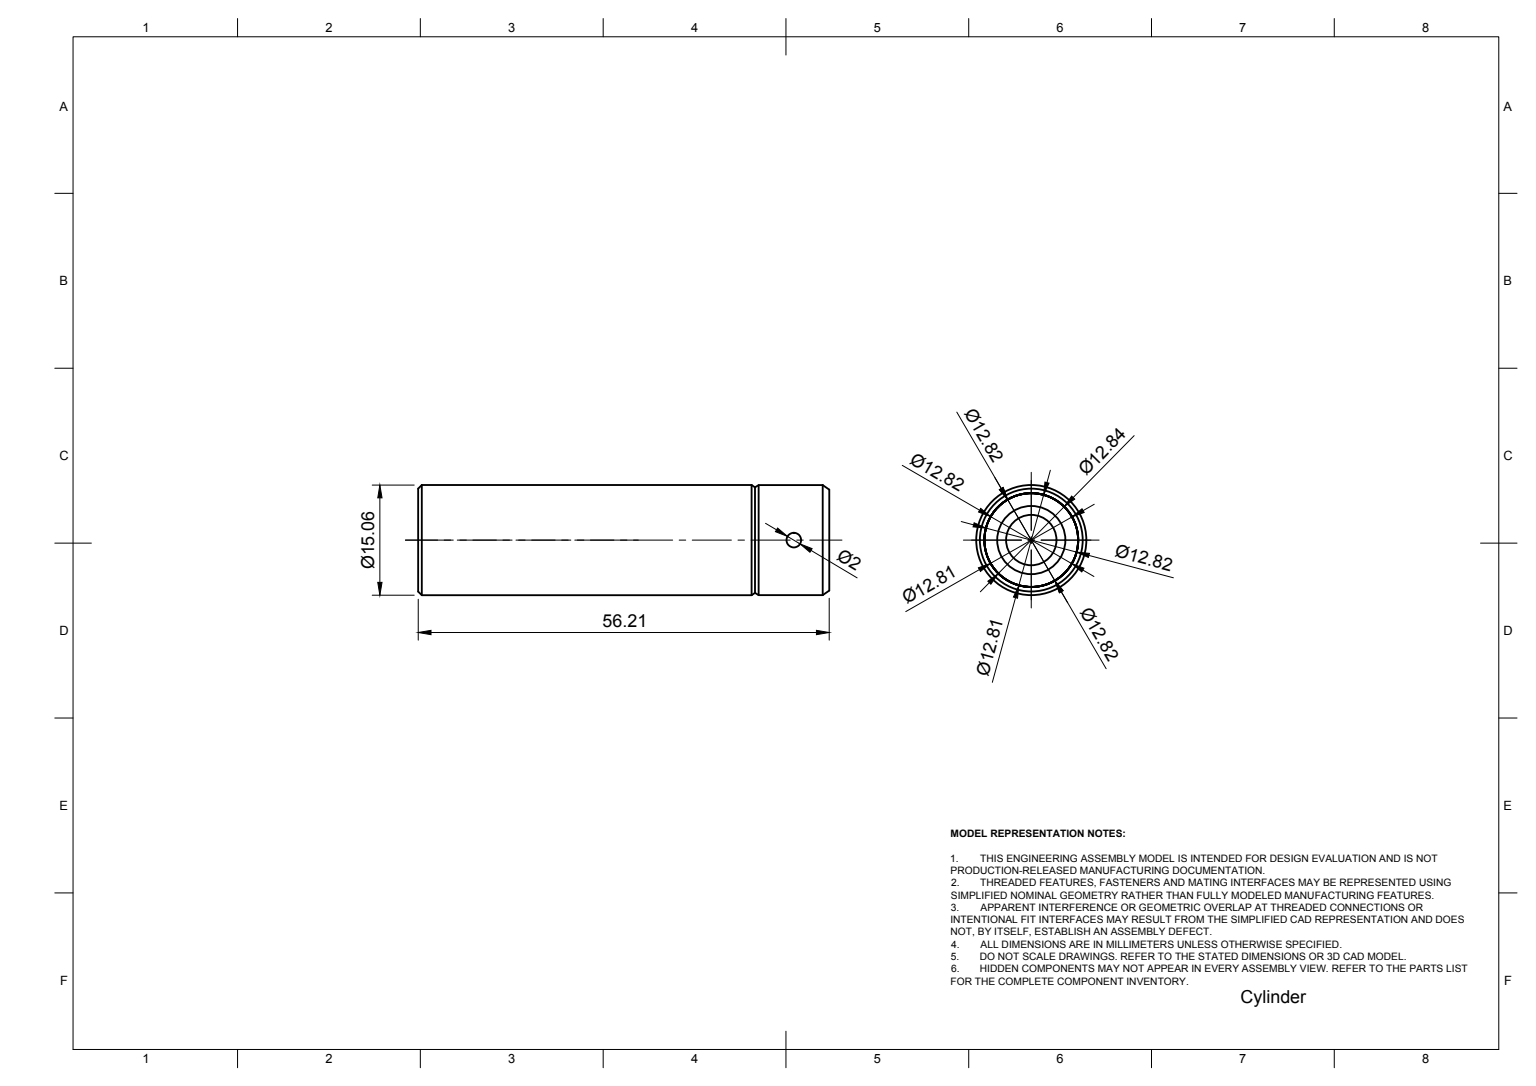
ISO-10303-21;
HEADER;
/* Generated by software containing ST-Developer
 * from STEP Tools, Inc. (www.steptools.com) 
 */

FILE_DESCRIPTION(
/* description */ (''),
/* implementation_level */ '2;1');

FILE_NAME(
/* name */ 'Cylinder.step',
/* time_stamp */ '2026-10-06T13:15:55-07:00',
/* author */ (''),
/* organization */ (''),
/* preprocessor_version */ 'ST-DEVELOPER v20.2',
/* originating_system */ 'Autodesk Translation Framework v15.15.0.0',
/* authorisation */ '');

FILE_SCHEMA (('AUTOMOTIVE_DESIGN { 1 0 10303 214 3 1 1 }'));
ENDSEC;

DATA;
#10=MECHANICAL_DESIGN_GEOMETRIC_PRESENTATION_REPRESENTATION('',(#114),#27707);
#73=CONICAL_SURFACE('',#4093,7.27835105742136,0.785398163397451);
#74=CONICAL_SURFACE('',#4106,7.20746054905241,0.610790367386849);
#75=CONICAL_SURFACE('',#4111,7.36529369971832,0.557210682142491);
#76=CONICAL_SURFACE('',#4113,7.36790580323689,0.610790367386849);
#77=CONICAL_SURFACE('',#4114,6.41628586403442,0.000295609290232646);
#78=CONICAL_SURFACE('',#4118,6.40906719549494,0.00029560929023293);
#79=CONICAL_SURFACE('',#4126,6.40820475053297,0.000295609290233083);
#80=CONICAL_SURFACE('',#4130,6.40732538114918,0.000295609290232334);
#81=CONICAL_SURFACE('',#4134,6.40667124022599,0.000295609290231853);
#94=SHAPE_REPRESENTATION_RELATIONSHIP('SRR','None',#27751,#104);
#104=ADVANCED_BREP_SHAPE_REPRESENTATION('',(#124),#27703);
#114=STYLED_ITEM('',(#27804),#124);
#124=MANIFOLD_SOLID_BREP('Body1',#3840);
#142=FACE_BOUND('',#796,.T.);
#143=FACE_BOUND('',#801,.T.);
#144=FACE_BOUND('',#804,.T.);
#145=FACE_BOUND('',#811,.T.);
#146=FACE_BOUND('',#814,.T.);
#147=FACE_BOUND('',#821,.T.);
#148=FACE_BOUND('',#824,.T.);
#149=FACE_BOUND('',#826,.T.);
#150=FACE_BOUND('',#828,.T.);
#194=PLANE('',#4096);
#195=PLANE('',#4104);
#196=PLANE('',#4120);
#197=PLANE('',#4124);
#198=PLANE('',#4136);
#199=PLANE('',#4140);
#200=PLANE('',#4143);
#260=CIRCLE('',#4094,7.52835105742136);
#261=CIRCLE('',#4095,7.02835105742136);
#262=CIRCLE('',#4097,6.42021067919505);
#263=CIRCLE('',#4099,7.52835105742136);
#264=CIRCLE('',#4102,5.);
#265=CIRCLE('',#4103,5.);
#266=CIRCLE('',#4105,3.44589712386029);
#267=CIRCLE('',#4107,7.52312685038423);
#268=CIRCLE('',#4108,6.89179424772059);
#269=CIRCLE('',#4110,7.52312685038423);
#270=CIRCLE('',#4112,7.20746054905241);
#271=CIRCLE('',#4115,6.40969108660508);
#272=CIRCLE('',#4117,6.40969108660508);
#273=CIRCLE('',#4119,6.40881029802658);
#274=CIRCLE('',#4121,6.41550316824698);
#275=CIRCLE('',#4123,6.41550316824698);
#276=CIRCLE('',#4125,6.40853872070288);
#277=CIRCLE('',#4127,6.40787078036307);
#278=CIRCLE('',#4129,6.40787078036307);
#279=CIRCLE('',#4131,6.40706623219228);
#280=CIRCLE('',#4133,6.40706623219228);
#281=CIRCLE('',#4135,6.4065967297173);
#282=CIRCLE('',#4137,4.66385643997278);
#283=CIRCLE('',#4139,4.66385643997278);
#284=CIRCLE('',#4141,3.44589712386029);
#393=CYLINDRICAL_SURFACE('',#4098,7.52835105742136);
#394=CYLINDRICAL_SURFACE('',#4100,0.999999999999999);
#395=CYLINDRICAL_SURFACE('',#4101,5.);
#396=CYLINDRICAL_SURFACE('',#4109,7.52312685038423);
#397=CYLINDRICAL_SURFACE('',#4116,6.40969108660508);
#398=CYLINDRICAL_SURFACE('',#4122,6.41550316824698);
#399=CYLINDRICAL_SURFACE('',#4128,6.40787078036307);
#400=CYLINDRICAL_SURFACE('',#4132,6.40706623219228);
#401=CYLINDRICAL_SURFACE('',#4138,4.66385643997278);
#402=CYLINDRICAL_SURFACE('',#4142,3.44589712386029);
#559=FACE_OUTER_BOUND('',#794,.T.);
#560=FACE_OUTER_BOUND('',#795,.T.);
#561=FACE_OUTER_BOUND('',#797,.T.);
#562=FACE_OUTER_BOUND('',#798,.T.);
#563=FACE_OUTER_BOUND('',#799,.T.);
#564=FACE_OUTER_BOUND('',#800,.T.);
#565=FACE_OUTER_BOUND('',#802,.T.);
#566=FACE_OUTER_BOUND('',#803,.T.);
#567=FACE_OUTER_BOUND('',#805,.T.);
#568=FACE_OUTER_BOUND('',#806,.T.);
#569=FACE_OUTER_BOUND('',#807,.T.);
#570=FACE_OUTER_BOUND('',#808,.T.);
#571=FACE_OUTER_BOUND('',#809,.T.);
#572=FACE_OUTER_BOUND('',#810,.T.);
#573=FACE_OUTER_BOUND('',#812,.T.);
#574=FACE_OUTER_BOUND('',#813,.T.);
#575=FACE_OUTER_BOUND('',#815,.T.);
#576=FACE_OUTER_BOUND('',#816,.T.);
#577=FACE_OUTER_BOUND('',#817,.T.);
#578=FACE_OUTER_BOUND('',#818,.T.);
#579=FACE_OUTER_BOUND('',#819,.T.);
#580=FACE_OUTER_BOUND('',#820,.T.);
#581=FACE_OUTER_BOUND('',#822,.T.);
#582=FACE_OUTER_BOUND('',#823,.T.);
#583=FACE_OUTER_BOUND('',#825,.T.);
#584=FACE_OUTER_BOUND('',#827,.T.);
#794=EDGE_LOOP('',(#3123,#3124,#3125,#3126));
#795=EDGE_LOOP('',(#3127));
#796=EDGE_LOOP('',(#3128));
#797=EDGE_LOOP('',(#3129,#3130,#3131,#3132));
#798=EDGE_LOOP('',(#3133,#3134,#3135,#3136,#3137,#3138));
#799=EDGE_LOOP('',(#3139,#3140,#3141,#3142));
#800=EDGE_LOOP('',(#3143));
#801=EDGE_LOOP('',(#3144));
#802=EDGE_LOOP('',(#3145,#3146,#3147,#3148));
#803=EDGE_LOOP('',(#3149,#3150,#3151,#3152));
#804=EDGE_LOOP('',(#3153,#3154));
#805=EDGE_LOOP('',(#3155,#3156,#3157,#3158));
#806=EDGE_LOOP('',(#3159,#3160,#3161,#3162));
#807=EDGE_LOOP('',(#3163,#3164,#3165,#3166));
#808=EDGE_LOOP('',(#3167,#3168,#3169,#3170));
#809=EDGE_LOOP('',(#3171,#3172,#3173,#3174));
#810=EDGE_LOOP('',(#3175));
#811=EDGE_LOOP('',(#3176));
#812=EDGE_LOOP('',(#3177,#3178,#3179,#3180));
#813=EDGE_LOOP('',(#3181));
#814=EDGE_LOOP('',(#3182));
#815=EDGE_LOOP('',(#3183,#3184,#3185,#3186));
#816=EDGE_LOOP('',(#3187,#3188,#3189,#3190));
#817=EDGE_LOOP('',(#3191,#3192,#3193,#3194));
#818=EDGE_LOOP('',(#3195,#3196,#3197,#3198));
#819=EDGE_LOOP('',(#3199,#3200,#3201,#3202));
#820=EDGE_LOOP('',(#3203));
#821=EDGE_LOOP('',(#3204));
#822=EDGE_LOOP('',(#3205,#3206,#3207,#3208));
#823=EDGE_LOOP('',(#3209));
#824=EDGE_LOOP('',(#3210));
#825=EDGE_LOOP('',(#3211,#3212,#3213,#3214));
#826=EDGE_LOOP('',(#3215,#3216));
#827=EDGE_LOOP('',(#3217));
#828=EDGE_LOOP('',(#3218));
#1032=LINE('',#15534,#1208);
#1033=LINE('',#15541,#1209);
#1034=LINE('',#15583,#1210);
#1035=LINE('',#15625,#1211);
#1036=LINE('',#15634,#1212);
#1037=LINE('',#15639,#1213);
#1038=LINE('',#15642,#1214);
#1039=LINE('',#15645,#1215);
#1040=LINE('',#15649,#1216);
#1041=LINE('',#15653,#1217);
#1042=LINE('',#15657,#1218);
#1043=LINE('',#15664,#1219);
#1044=LINE('',#15671,#1220);
#1045=LINE('',#15675,#1221);
#1046=LINE('',#15679,#1222);
#1047=LINE('',#15683,#1223);
#1048=LINE('',#15687,#1224);
#1049=LINE('',#15694,#1225);
#1050=LINE('',#15699,#1226);
#1208=VECTOR('',#4685,7.27835105742136);
#1209=VECTOR('',#4694,7.52835105742136);
#1210=VECTOR('',#4699,0.999999999999999);
#1211=VECTOR('',#4704,5.);
#1212=VECTOR('',#4715,7.20746054905241);
#1213=VECTOR('',#4722,7.52312685038423);
#1214=VECTOR('',#4725,7.36529369971832);
#1215=VECTOR('',#4730,7.36790580323689);
#1216=VECTOR('',#4735,6.41628586403442);
#1217=VECTOR('',#4740,6.40969108660508);
#1218=VECTOR('',#4745,6.40906719549494);
#1219=VECTOR('',#4754,6.41550316824698);
#1220=VECTOR('',#4763,6.40820475053297);
#1221=VECTOR('',#4768,6.40787078036307);
#1222=VECTOR('',#4773,6.40732538114918);
#1223=VECTOR('',#4778,6.40706623219228);
#1224=VECTOR('',#4783,6.40667124022599);
#1225=VECTOR('',#4792,4.66385643997278);
#1226=VECTOR('',#4799,3.44589712386029);
#1438=B_SPLINE_CURVE_WITH_KNOTS('',3,(#15546,#15547,#15548,#15549,#15550,
#15551,#15552,#15553,#15554,#15555,#15556,#15557,#15558,#15559,#15560,#15561,
#15562,#15563,#15564,#15565,#15566,#15567,#15568,#15569,#15570,#15571),
 .UNSPECIFIED.,.F.,.F.,(4,2,2,2,2,2,2,2,2,2,2,2,4),(-0.606481282784619,
-0.568571286664201,-0.530661290543783,-0.492761126316124,-0.454860962088464,
-0.416960797860805,-0.379060633633146,-0.341150637512728,-0.30324064139231,
-0.265330645271891,-0.227420649151473,-0.189520484923814,-0.151620320696155),
 .UNSPECIFIED.);
#1439=B_SPLINE_CURVE_WITH_KNOTS('',3,(#15572,#15573,#15574,#15575,#15576,
#15577,#15578,#15579,#15580,#15581),.UNSPECIFIED.,.F.,.F.,(4,2,2,2,4),(-0.151620320696155,
-0.113720156468496,-0.0758199922408364,-0.0379099961204182,0.),
 .UNSPECIFIED.);
#1440=B_SPLINE_CURVE_WITH_KNOTS('',3,(#15585,#15586,#15587,#15588,#15589,
#15590,#15591,#15592,#15593,#15594),.UNSPECIFIED.,.F.,.F.,(4,2,2,2,4),(0.,
0.0377168406459521,0.0754336812919042,0.113150118256495,0.150866555221085),
 .UNSPECIFIED.);
#1441=B_SPLINE_CURVE_WITH_KNOTS('',3,(#15595,#15596,#15597,#15598,#15599,
#15600,#15601,#15602,#15603,#15604,#15605,#15606,#15607,#15608,#15609,#15610,
#15611,#15612,#15613,#15614,#15615,#15616,#15617,#15618,#15619,#15620),
 .UNSPECIFIED.,.F.,.F.,(4,2,2,2,2,2,2,2,2,2,2,2,4),(0.150866555221085,0.188582992185676,
0.226299429150267,0.264016269796219,0.301733110442171,0.339449951088123,
0.377166791734075,0.414883228698666,0.452599665663256,0.490316102627847,
0.528032539592437,0.565749380238389,0.603466220884342),.UNSPECIFIED.);
#1749=VERTEX_POINT('',#15531);
#1750=VERTEX_POINT('',#15533);
#1751=VERTEX_POINT('',#15537);
#1752=VERTEX_POINT('',#15540);
#1753=VERTEX_POINT('',#15544);
#1754=VERTEX_POINT('',#15545);
#1755=VERTEX_POINT('',#15582);
#1756=VERTEX_POINT('',#15584);
#1757=VERTEX_POINT('',#15622);
#1758=VERTEX_POINT('',#15624);
#1759=VERTEX_POINT('',#15628);
#1760=VERTEX_POINT('',#15631);
#1761=VERTEX_POINT('',#15633);
#1762=VERTEX_POINT('',#15637);
#1763=VERTEX_POINT('',#15641);
#1764=VERTEX_POINT('',#15647);
#1765=VERTEX_POINT('',#15651);
#1766=VERTEX_POINT('',#15655);
#1767=VERTEX_POINT('',#15659);
#1768=VERTEX_POINT('',#15662);
#1769=VERTEX_POINT('',#15666);
#1770=VERTEX_POINT('',#15669);
#1771=VERTEX_POINT('',#15673);
#1772=VERTEX_POINT('',#15677);
#1773=VERTEX_POINT('',#15681);
#1774=VERTEX_POINT('',#15685);
#1775=VERTEX_POINT('',#15689);
#1776=VERTEX_POINT('',#15692);
#1777=VERTEX_POINT('',#15696);
#2231=EDGE_CURVE('',#1749,#1749,#260,.T.);
#2232=EDGE_CURVE('',#1749,#1750,#1032,.T.);
#2233=EDGE_CURVE('',#1750,#1750,#261,.T.);
#2234=EDGE_CURVE('',#1751,#1751,#262,.T.);
#2235=EDGE_CURVE('',#1749,#1752,#1033,.T.);
#2236=EDGE_CURVE('',#1752,#1752,#263,.T.);
#2237=EDGE_CURVE('',#1753,#1754,#1438,.T.);
#2238=EDGE_CURVE('',#1754,#1753,#1439,.T.);
#2239=EDGE_CURVE('',#1754,#1755,#1034,.T.);
#2240=EDGE_CURVE('',#1756,#1755,#1440,.T.);
#2241=EDGE_CURVE('',#1755,#1756,#1441,.T.);
#2242=EDGE_CURVE('',#1757,#1757,#264,.T.);
#2243=EDGE_CURVE('',#1757,#1758,#1035,.T.);
#2244=EDGE_CURVE('',#1758,#1758,#265,.T.);
#2245=EDGE_CURVE('',#1759,#1759,#266,.T.);
#2246=EDGE_CURVE('',#1760,#1760,#267,.T.);
#2247=EDGE_CURVE('',#1760,#1761,#1036,.T.);
#2248=EDGE_CURVE('',#1761,#1761,#268,.T.);
#2249=EDGE_CURVE('',#1762,#1762,#269,.T.);
#2250=EDGE_CURVE('',#1762,#1760,#1037,.T.);
#2251=EDGE_CURVE('',#1762,#1763,#1038,.T.);
#2252=EDGE_CURVE('',#1763,#1763,#270,.T.);
#2253=EDGE_CURVE('',#1752,#1763,#1039,.T.);
#2254=EDGE_CURVE('',#1764,#1764,#271,.T.);
#2255=EDGE_CURVE('',#1764,#1751,#1040,.T.);
#2256=EDGE_CURVE('',#1765,#1765,#272,.T.);
#2257=EDGE_CURVE('',#1765,#1764,#1041,.T.);
#2258=EDGE_CURVE('',#1766,#1766,#273,.T.);
#2259=EDGE_CURVE('',#1766,#1765,#1042,.T.);
#2260=EDGE_CURVE('',#1767,#1767,#274,.T.);
#2261=EDGE_CURVE('',#1768,#1768,#275,.T.);
#2262=EDGE_CURVE('',#1768,#1767,#1043,.T.);
#2263=EDGE_CURVE('',#1769,#1769,#276,.T.);
#2264=EDGE_CURVE('',#1770,#1770,#277,.T.);
#2265=EDGE_CURVE('',#1770,#1769,#1044,.T.);
#2266=EDGE_CURVE('',#1771,#1771,#278,.T.);
#2267=EDGE_CURVE('',#1771,#1770,#1045,.T.);
#2268=EDGE_CURVE('',#1772,#1772,#279,.T.);
#2269=EDGE_CURVE('',#1772,#1771,#1046,.T.);
#2270=EDGE_CURVE('',#1773,#1773,#280,.T.);
#2271=EDGE_CURVE('',#1773,#1772,#1047,.T.);
#2272=EDGE_CURVE('',#1774,#1774,#281,.T.);
#2273=EDGE_CURVE('',#1774,#1773,#1048,.T.);
#2274=EDGE_CURVE('',#1775,#1775,#282,.T.);
#2275=EDGE_CURVE('',#1776,#1776,#283,.T.);
#2276=EDGE_CURVE('',#1776,#1775,#1049,.T.);
#2277=EDGE_CURVE('',#1777,#1777,#284,.T.);
#2278=EDGE_CURVE('',#1759,#1777,#1050,.T.);
#3123=ORIENTED_EDGE('',*,*,#2231,.T.);
#3124=ORIENTED_EDGE('',*,*,#2232,.T.);
#3125=ORIENTED_EDGE('',*,*,#2233,.T.);
#3126=ORIENTED_EDGE('',*,*,#2232,.F.);
#3127=ORIENTED_EDGE('',*,*,#2233,.F.);
#3128=ORIENTED_EDGE('',*,*,#2234,.F.);
#3129=ORIENTED_EDGE('',*,*,#2231,.F.);
#3130=ORIENTED_EDGE('',*,*,#2235,.T.);
#3131=ORIENTED_EDGE('',*,*,#2236,.T.);
#3132=ORIENTED_EDGE('',*,*,#2235,.F.);
#3133=ORIENTED_EDGE('',*,*,#2237,.F.);
#3134=ORIENTED_EDGE('',*,*,#2238,.F.);
#3135=ORIENTED_EDGE('',*,*,#2239,.T.);
#3136=ORIENTED_EDGE('',*,*,#2240,.F.);
#3137=ORIENTED_EDGE('',*,*,#2241,.F.);
#3138=ORIENTED_EDGE('',*,*,#2239,.F.);
#3139=ORIENTED_EDGE('',*,*,#2242,.F.);
#3140=ORIENTED_EDGE('',*,*,#2243,.T.);
#3141=ORIENTED_EDGE('',*,*,#2244,.T.);
#3142=ORIENTED_EDGE('',*,*,#2243,.F.);
#3143=ORIENTED_EDGE('',*,*,#2244,.F.);
#3144=ORIENTED_EDGE('',*,*,#2245,.T.);
#3145=ORIENTED_EDGE('',*,*,#2246,.F.);
#3146=ORIENTED_EDGE('',*,*,#2247,.T.);
#3147=ORIENTED_EDGE('',*,*,#2248,.T.);
#3148=ORIENTED_EDGE('',*,*,#2247,.F.);
#3149=ORIENTED_EDGE('',*,*,#2249,.F.);
#3150=ORIENTED_EDGE('',*,*,#2250,.T.);
#3151=ORIENTED_EDGE('',*,*,#2246,.T.);
#3152=ORIENTED_EDGE('',*,*,#2250,.F.);
#3153=ORIENTED_EDGE('',*,*,#2240,.T.);
#3154=ORIENTED_EDGE('',*,*,#2241,.T.);
#3155=ORIENTED_EDGE('',*,*,#2249,.T.);
#3156=ORIENTED_EDGE('',*,*,#2251,.T.);
#3157=ORIENTED_EDGE('',*,*,#2252,.F.);
#3158=ORIENTED_EDGE('',*,*,#2251,.F.);
#3159=ORIENTED_EDGE('',*,*,#2236,.F.);
#3160=ORIENTED_EDGE('',*,*,#2253,.T.);
#3161=ORIENTED_EDGE('',*,*,#2252,.T.);
#3162=ORIENTED_EDGE('',*,*,#2253,.F.);
#3163=ORIENTED_EDGE('',*,*,#2254,.F.);
#3164=ORIENTED_EDGE('',*,*,#2255,.T.);
#3165=ORIENTED_EDGE('',*,*,#2234,.T.);
#3166=ORIENTED_EDGE('',*,*,#2255,.F.);
#3167=ORIENTED_EDGE('',*,*,#2256,.F.);
#3168=ORIENTED_EDGE('',*,*,#2257,.T.);
#3169=ORIENTED_EDGE('',*,*,#2254,.T.);
#3170=ORIENTED_EDGE('',*,*,#2257,.F.);
#3171=ORIENTED_EDGE('',*,*,#2258,.F.);
#3172=ORIENTED_EDGE('',*,*,#2259,.T.);
#3173=ORIENTED_EDGE('',*,*,#2256,.T.);
#3174=ORIENTED_EDGE('',*,*,#2259,.F.);
#3175=ORIENTED_EDGE('',*,*,#2260,.F.);
#3176=ORIENTED_EDGE('',*,*,#2258,.T.);
#3177=ORIENTED_EDGE('',*,*,#2261,.F.);
#3178=ORIENTED_EDGE('',*,*,#2262,.T.);
#3179=ORIENTED_EDGE('',*,*,#2260,.T.);
#3180=ORIENTED_EDGE('',*,*,#2262,.F.);
#3181=ORIENTED_EDGE('',*,*,#2261,.T.);
#3182=ORIENTED_EDGE('',*,*,#2263,.F.);
#3183=ORIENTED_EDGE('',*,*,#2264,.F.);
#3184=ORIENTED_EDGE('',*,*,#2265,.T.);
#3185=ORIENTED_EDGE('',*,*,#2263,.T.);
#3186=ORIENTED_EDGE('',*,*,#2265,.F.);
#3187=ORIENTED_EDGE('',*,*,#2266,.F.);
#3188=ORIENTED_EDGE('',*,*,#2267,.T.);
#3189=ORIENTED_EDGE('',*,*,#2264,.T.);
#3190=ORIENTED_EDGE('',*,*,#2267,.F.);
#3191=ORIENTED_EDGE('',*,*,#2268,.F.);
#3192=ORIENTED_EDGE('',*,*,#2269,.T.);
#3193=ORIENTED_EDGE('',*,*,#2266,.T.);
#3194=ORIENTED_EDGE('',*,*,#2269,.F.);
#3195=ORIENTED_EDGE('',*,*,#2270,.F.);
#3196=ORIENTED_EDGE('',*,*,#2271,.T.);
#3197=ORIENTED_EDGE('',*,*,#2268,.T.);
#3198=ORIENTED_EDGE('',*,*,#2271,.F.);
#3199=ORIENTED_EDGE('',*,*,#2272,.F.);
#3200=ORIENTED_EDGE('',*,*,#2273,.T.);
#3201=ORIENTED_EDGE('',*,*,#2270,.T.);
#3202=ORIENTED_EDGE('',*,*,#2273,.F.);
#3203=ORIENTED_EDGE('',*,*,#2272,.T.);
#3204=ORIENTED_EDGE('',*,*,#2274,.F.);
#3205=ORIENTED_EDGE('',*,*,#2275,.F.);
#3206=ORIENTED_EDGE('',*,*,#2276,.T.);
#3207=ORIENTED_EDGE('',*,*,#2274,.T.);
#3208=ORIENTED_EDGE('',*,*,#2276,.F.);
#3209=ORIENTED_EDGE('',*,*,#2275,.T.);
#3210=ORIENTED_EDGE('',*,*,#2277,.F.);
#3211=ORIENTED_EDGE('',*,*,#2245,.F.);
#3212=ORIENTED_EDGE('',*,*,#2278,.T.);
#3213=ORIENTED_EDGE('',*,*,#2277,.T.);
#3214=ORIENTED_EDGE('',*,*,#2278,.F.);
#3215=ORIENTED_EDGE('',*,*,#2237,.T.);
#3216=ORIENTED_EDGE('',*,*,#2238,.T.);
#3217=ORIENTED_EDGE('',*,*,#2248,.F.);
#3218=ORIENTED_EDGE('',*,*,#2242,.T.);
#3734=ADVANCED_FACE('',(#559),#73,.T.);
#3735=ADVANCED_FACE('',(#560,#142),#194,.F.);
#3736=ADVANCED_FACE('',(#561),#393,.T.);
#3737=ADVANCED_FACE('',(#562),#394,.F.);
#3738=ADVANCED_FACE('',(#563),#395,.F.);
#3739=ADVANCED_FACE('',(#564,#143),#195,.T.);
#3740=ADVANCED_FACE('',(#565),#74,.T.);
#3741=ADVANCED_FACE('',(#566,#144),#396,.T.);
#3742=ADVANCED_FACE('',(#567),#75,.T.);
#3743=ADVANCED_FACE('',(#568),#76,.T.);
#3744=ADVANCED_FACE('',(#569),#77,.F.);
#3745=ADVANCED_FACE('',(#570),#397,.F.);
#3746=ADVANCED_FACE('',(#571),#78,.F.);
#3747=ADVANCED_FACE('',(#572,#145),#196,.T.);
#3748=ADVANCED_FACE('',(#573),#398,.F.);
#3749=ADVANCED_FACE('',(#574,#146),#197,.T.);
#3750=ADVANCED_FACE('',(#575),#79,.F.);
#3751=ADVANCED_FACE('',(#576),#399,.F.);
#3752=ADVANCED_FACE('',(#577),#80,.F.);
#3753=ADVANCED_FACE('',(#578),#400,.F.);
#3754=ADVANCED_FACE('',(#579),#81,.F.);
#3755=ADVANCED_FACE('',(#580,#147),#198,.T.);
#3756=ADVANCED_FACE('',(#581),#401,.F.);
#3757=ADVANCED_FACE('',(#582,#148),#199,.T.);
#3758=ADVANCED_FACE('',(#583,#149),#402,.F.);
#3759=ADVANCED_FACE('',(#584,#150),#200,.T.);
#3840=CLOSED_SHELL('',(#3734,#3735,#3736,#3737,#3738,#3739,#3740,#3741,
#3742,#3743,#3744,#3745,#3746,#3747,#3748,#3749,#3750,#3751,#3752,#3753,
#3754,#3755,#3756,#3757,#3758,#3759));
#4092=AXIS2_PLACEMENT_3D('',#15529,#4679,#4680);
#4093=AXIS2_PLACEMENT_3D('',#15530,#4681,#4682);
#4094=AXIS2_PLACEMENT_3D('',#15532,#4683,#4684);
#4095=AXIS2_PLACEMENT_3D('',#15535,#4686,#4687);
#4096=AXIS2_PLACEMENT_3D('',#15536,#4688,#4689);
#4097=AXIS2_PLACEMENT_3D('',#15538,#4690,#4691);
#4098=AXIS2_PLACEMENT_3D('',#15539,#4692,#4693);
#4099=AXIS2_PLACEMENT_3D('',#15542,#4695,#4696);
#4100=AXIS2_PLACEMENT_3D('',#15543,#4697,#4698);
#4101=AXIS2_PLACEMENT_3D('',#15621,#4700,#4701);
#4102=AXIS2_PLACEMENT_3D('',#15623,#4702,#4703);
#4103=AXIS2_PLACEMENT_3D('',#15626,#4705,#4706);
#4104=AXIS2_PLACEMENT_3D('',#15627,#4707,#4708);
#4105=AXIS2_PLACEMENT_3D('',#15629,#4709,#4710);
#4106=AXIS2_PLACEMENT_3D('',#15630,#4711,#4712);
#4107=AXIS2_PLACEMENT_3D('',#15632,#4713,#4714);
#4108=AXIS2_PLACEMENT_3D('',#15635,#4716,#4717);
#4109=AXIS2_PLACEMENT_3D('',#15636,#4718,#4719);
#4110=AXIS2_PLACEMENT_3D('',#15638,#4720,#4721);
#4111=AXIS2_PLACEMENT_3D('',#15640,#4723,#4724);
#4112=AXIS2_PLACEMENT_3D('',#15643,#4726,#4727);
#4113=AXIS2_PLACEMENT_3D('',#15644,#4728,#4729);
#4114=AXIS2_PLACEMENT_3D('',#15646,#4731,#4732);
#4115=AXIS2_PLACEMENT_3D('',#15648,#4733,#4734);
#4116=AXIS2_PLACEMENT_3D('',#15650,#4736,#4737);
#4117=AXIS2_PLACEMENT_3D('',#15652,#4738,#4739);
#4118=AXIS2_PLACEMENT_3D('',#15654,#4741,#4742);
#4119=AXIS2_PLACEMENT_3D('',#15656,#4743,#4744);
#4120=AXIS2_PLACEMENT_3D('',#15658,#4746,#4747);
#4121=AXIS2_PLACEMENT_3D('',#15660,#4748,#4749);
#4122=AXIS2_PLACEMENT_3D('',#15661,#4750,#4751);
#4123=AXIS2_PLACEMENT_3D('',#15663,#4752,#4753);
#4124=AXIS2_PLACEMENT_3D('',#15665,#4755,#4756);
#4125=AXIS2_PLACEMENT_3D('',#15667,#4757,#4758);
#4126=AXIS2_PLACEMENT_3D('',#15668,#4759,#4760);
#4127=AXIS2_PLACEMENT_3D('',#15670,#4761,#4762);
#4128=AXIS2_PLACEMENT_3D('',#15672,#4764,#4765);
#4129=AXIS2_PLACEMENT_3D('',#15674,#4766,#4767);
#4130=AXIS2_PLACEMENT_3D('',#15676,#4769,#4770);
#4131=AXIS2_PLACEMENT_3D('',#15678,#4771,#4772);
#4132=AXIS2_PLACEMENT_3D('',#15680,#4774,#4775);
#4133=AXIS2_PLACEMENT_3D('',#15682,#4776,#4777);
#4134=AXIS2_PLACEMENT_3D('',#15684,#4779,#4780);
#4135=AXIS2_PLACEMENT_3D('',#15686,#4781,#4782);
#4136=AXIS2_PLACEMENT_3D('',#15688,#4784,#4785);
#4137=AXIS2_PLACEMENT_3D('',#15690,#4786,#4787);
#4138=AXIS2_PLACEMENT_3D('',#15691,#4788,#4789);
#4139=AXIS2_PLACEMENT_3D('',#15693,#4790,#4791);
#4140=AXIS2_PLACEMENT_3D('',#15695,#4793,#4794);
#4141=AXIS2_PLACEMENT_3D('',#15697,#4795,#4796);
#4142=AXIS2_PLACEMENT_3D('',#15698,#4797,#4798);
#4143=AXIS2_PLACEMENT_3D('',#15700,#4800,#4801);
#4679=DIRECTION('axis',(0.,0.,1.));
#4680=DIRECTION('refdir',(1.,0.,0.));
#4681=DIRECTION('center_axis',(-1.,0.,0.));
#4682=DIRECTION('ref_axis',(0.,0.,-1.));
#4683=DIRECTION('center_axis',(1.,0.,0.));
#4684=DIRECTION('ref_axis',(0.,0.,-1.));
#4685=DIRECTION('',(0.707106781186546,-8.65956056235496E-17,-0.707106781186549));
#4686=DIRECTION('center_axis',(-1.,0.,0.));
#4687=DIRECTION('ref_axis',(0.,0.,-1.));
#4688=DIRECTION('center_axis',(-1.,0.,0.));
#4689=DIRECTION('ref_axis',(0.,0.,1.));
#4690=DIRECTION('center_axis',(1.,0.,0.));
#4691=DIRECTION('ref_axis',(0.,0.,-1.));
#4692=DIRECTION('center_axis',(1.,0.,0.));
#4693=DIRECTION('ref_axis',(0.,0.,-1.));
#4694=DIRECTION('',(-1.,0.,0.));
#4695=DIRECTION('center_axis',(1.,0.,0.));
#4696=DIRECTION('ref_axis',(0.,0.,-1.));
#4697=DIRECTION('center_axis',(0.,1.,0.));
#4698=DIRECTION('ref_axis',(1.,0.,0.));
#4699=DIRECTION('',(0.,1.,0.));
#4700=DIRECTION('center_axis',(1.,0.,0.));
#4701=DIRECTION('ref_axis',(0.,-1.,0.));
#4702=DIRECTION('center_axis',(1.,0.,0.));
#4703=DIRECTION('ref_axis',(0.,-1.,0.));
#4704=DIRECTION('',(1.,0.,0.));
#4705=DIRECTION('center_axis',(1.,0.,0.));
#4706=DIRECTION('ref_axis',(0.,-1.,0.));
#4707=DIRECTION('center_axis',(-1.,0.,0.));
#4708=DIRECTION('ref_axis',(0.,-1.,0.));
#4709=DIRECTION('center_axis',(1.,0.,0.));
#4710=DIRECTION('ref_axis',(0.,0.,-1.));
#4711=DIRECTION('center_axis',(1.,0.,0.));
#4712=DIRECTION('ref_axis',(0.,0.,-1.));
#4713=DIRECTION('center_axis',(1.,0.,0.));
#4714=DIRECTION('ref_axis',(0.,0.,-1.));
#4715=DIRECTION('',(-0.819194986126072,7.02353436578877E-17,-0.573515104165448));
#4716=DIRECTION('center_axis',(1.,0.,0.));
#4717=DIRECTION('ref_axis',(0.,0.,-1.));
#4718=DIRECTION('center_axis',(1.,0.,0.));
#4719=DIRECTION('ref_axis',(0.,0.,-1.));
#4720=DIRECTION('center_axis',(1.,0.,0.));
#4721=DIRECTION('ref_axis',(0.,0.,-1.));
#4722=DIRECTION('',(-1.,0.,0.));
#4723=DIRECTION('center_axis',(-1.,0.,0.));
#4724=DIRECTION('ref_axis',(0.,0.,-1.));
#4725=DIRECTION('',(0.848733460294827,-6.47618786727041E-17,-0.528820870783264));
#4726=DIRECTION('center_axis',(1.,0.,0.));
#4727=DIRECTION('ref_axis',(0.,0.,-1.));
#4728=DIRECTION('center_axis',(1.,0.,0.));
#4729=DIRECTION('ref_axis',(0.,0.,-1.));
#4730=DIRECTION('',(-0.819194986126072,7.02353436578877E-17,-0.573515104165448));
#4731=DIRECTION('center_axis',(1.,0.,0.));
#4732=DIRECTION('ref_axis',(0.,0.,-1.));
#4733=DIRECTION('center_axis',(1.,0.,0.));
#4734=DIRECTION('ref_axis',(0.,0.,-1.));
#4735=DIRECTION('',(0.999999956307574,-3.62016965809164E-20,0.00029560928592735));
#4736=DIRECTION('center_axis',(1.,0.,0.));
#4737=DIRECTION('ref_axis',(0.,0.,-1.));
#4738=DIRECTION('center_axis',(1.,0.,0.));
#4739=DIRECTION('ref_axis',(0.,0.,-1.));
#4740=DIRECTION('',(1.,0.,0.));
#4741=DIRECTION('center_axis',(1.,0.,0.));
#4742=DIRECTION('ref_axis',(0.,0.,-1.));
#4743=DIRECTION('center_axis',(1.,0.,0.));
#4744=DIRECTION('ref_axis',(0.,0.,-1.));
#4745=DIRECTION('',(0.999999956307574,-3.62016965809512E-20,0.000295609285927634));
#4746=DIRECTION('center_axis',(-1.,0.,0.));
#4747=DIRECTION('ref_axis',(0.,0.,1.));
#4748=DIRECTION('center_axis',(1.,0.,0.));
#4749=DIRECTION('ref_axis',(0.,0.,-1.));
#4750=DIRECTION('center_axis',(1.,0.,0.));
#4751=DIRECTION('ref_axis',(0.,0.,-1.));
#4752=DIRECTION('center_axis',(1.,0.,0.));
#4753=DIRECTION('ref_axis',(0.,0.,-1.));
#4754=DIRECTION('',(1.,0.,0.));
#4755=DIRECTION('center_axis',(1.,0.,0.));
#4756=DIRECTION('ref_axis',(0.,0.,-1.));
#4757=DIRECTION('center_axis',(1.,0.,0.));
#4758=DIRECTION('ref_axis',(0.,0.,-1.));
#4759=DIRECTION('center_axis',(1.,0.,0.));
#4760=DIRECTION('ref_axis',(0.,0.,-1.));
#4761=DIRECTION('center_axis',(1.,0.,0.));
#4762=DIRECTION('ref_axis',(0.,0.,-1.));
#4763=DIRECTION('',(0.999999956307574,-3.62016965809699E-20,0.000295609285927787));
#4764=DIRECTION('center_axis',(1.,0.,0.));
#4765=DIRECTION('ref_axis',(0.,0.,-1.));
#4766=DIRECTION('center_axis',(1.,0.,0.));
#4767=DIRECTION('ref_axis',(0.,0.,-1.));
#4768=DIRECTION('',(1.,0.,0.));
#4769=DIRECTION('center_axis',(1.,0.,0.));
#4770=DIRECTION('ref_axis',(0.,0.,-1.));
#4771=DIRECTION('center_axis',(1.,0.,0.));
#4772=DIRECTION('ref_axis',(0.,0.,-1.));
#4773=DIRECTION('',(0.999999956307574,-3.62016965808782E-20,0.000295609285927038));
#4774=DIRECTION('center_axis',(1.,0.,0.));
#4775=DIRECTION('ref_axis',(0.,0.,-1.));
#4776=DIRECTION('center_axis',(1.,0.,0.));
#4777=DIRECTION('ref_axis',(0.,0.,-1.));
#4778=DIRECTION('',(1.,0.,0.));
#4779=DIRECTION('center_axis',(1.,0.,0.));
#4780=DIRECTION('ref_axis',(0.,0.,-1.));
#4781=DIRECTION('center_axis',(1.,0.,0.));
#4782=DIRECTION('ref_axis',(0.,0.,-1.));
#4783=DIRECTION('',(0.999999956307574,-3.62016965808193E-20,0.000295609285926557));
#4784=DIRECTION('center_axis',(1.,0.,0.));
#4785=DIRECTION('ref_axis',(0.,0.,-1.));
#4786=DIRECTION('center_axis',(1.,0.,0.));
#4787=DIRECTION('ref_axis',(0.,0.,-1.));
#4788=DIRECTION('center_axis',(1.,0.,0.));
#4789=DIRECTION('ref_axis',(0.,0.,-1.));
#4790=DIRECTION('center_axis',(1.,0.,0.));
#4791=DIRECTION('ref_axis',(0.,0.,-1.));
#4792=DIRECTION('',(1.,0.,0.));
#4793=DIRECTION('center_axis',(1.,0.,0.));
#4794=DIRECTION('ref_axis',(0.,0.,-1.));
#4795=DIRECTION('center_axis',(1.,0.,0.));
#4796=DIRECTION('ref_axis',(0.,0.,-1.));
#4797=DIRECTION('center_axis',(1.,0.,0.));
#4798=DIRECTION('ref_axis',(0.,0.,-1.));
#4799=DIRECTION('',(1.,0.,0.));
#4800=DIRECTION('center_axis',(-1.,0.,0.));
#4801=DIRECTION('ref_axis',(0.,0.,1.));
#15529=CARTESIAN_POINT('',(0.,0.,0.));
#15530=CARTESIAN_POINT('Origin',(66.9886855842388,0.,0.));
#15531=CARTESIAN_POINT('',(66.7386855842388,-9.21957102532866E-16,7.52835105742136));
#15532=CARTESIAN_POINT('Origin',(66.7386855842388,0.,0.));
#15533=CARTESIAN_POINT('',(67.2386855842388,8.60724762575498E-16,7.02835105742136));
#15534=CARTESIAN_POINT('',(66.9886855842388,8.91340932554182E-16,7.27835105742136));
#15535=CARTESIAN_POINT('Origin',(67.2386855842388,0.,0.));
#15536=CARTESIAN_POINT('Origin',(67.2386855842388,0.,-8.84759007750164));
#15537=CARTESIAN_POINT('',(67.2386855842388,-7.86249045812787E-16,6.42021067919505));
#15538=CARTESIAN_POINT('Origin',(67.2386855842388,0.,0.));
#15539=CARTESIAN_POINT('Origin',(48.2427605064424,0.,0.));
#15540=CARTESIAN_POINT('',(21.6431770351805,-9.21957102532866E-16,7.52835105742136));
#15541=CARTESIAN_POINT('',(48.2427605064424,-9.21957102532866E-16,7.52835105742136));
#15542=CARTESIAN_POINT('Origin',(21.6431770351805,0.,0.));
#15543=CARTESIAN_POINT('Origin',(15.8714473032184,0.,0.));
#15544=CARTESIAN_POINT('',(15.8714473032184,3.29760625124175,0.999999999999998));
#15545=CARTESIAN_POINT('',(14.8714473032184,3.44589712386029,-6.01983033610089E-17));
#15546=CARTESIAN_POINT('Ctrl Pts',(15.8714473032184,3.29760625124174,0.999999999999999));
#15547=CARTESIAN_POINT('Ctrl Pts',(15.9978139569531,3.29760625124174,0.999999999999999));
#15548=CARTESIAN_POINT('Ctrl Pts',(16.132068844028,3.30562953237115,0.974596096350375));
#15549=CARTESIAN_POINT('Ctrl Pts',(16.3782103010389,3.33407731229027,0.872325929581351));
#15550=CARTESIAN_POINT('Ctrl Pts',(16.4901654582252,3.3540348875684,0.795495407366277));
#15551=CARTESIAN_POINT('Ctrl Pts',(16.6669197871454,3.39109395594973,0.618741078446085));
#15552=CARTESIAN_POINT('Ctrl Pts',(16.7437680872924,3.41067812574963,0.506776556958312));
#15553=CARTESIAN_POINT('Ctrl Pts',(16.8460513462857,3.43826042485992,0.26060123975522));
#15554=CARTESIAN_POINT('Ctrl Pts',(16.8714473032184,3.44589712386029,0.126333880758864));
#15555=CARTESIAN_POINT('Ctrl Pts',(16.8714473032184,3.44589712386029,-0.126333880758864));
#15556=CARTESIAN_POINT('Ctrl Pts',(16.8460513462857,3.43826042485992,-0.260601239755222));
#15557=CARTESIAN_POINT('Ctrl Pts',(16.7437680872924,3.41067812574963,-0.506776556958312));
#15558=CARTESIAN_POINT('Ctrl Pts',(16.6669197871454,3.39109395594973,-0.618741078446085));
#15559=CARTESIAN_POINT('Ctrl Pts',(16.4901654582252,3.3540348875684,-0.795495407366277));
#15560=CARTESIAN_POINT('Ctrl Pts',(16.3782103010389,3.33407731229027,-0.872325929581349));
#15561=CARTESIAN_POINT('Ctrl Pts',(16.132068844028,3.30562953237115,-0.974596096350375));
#15562=CARTESIAN_POINT('Ctrl Pts',(15.9978139569531,3.29760625124174,-0.999999999999999));
#15563=CARTESIAN_POINT('Ctrl Pts',(15.7450806494837,3.29760625124174,-0.999999999999999));
#15564=CARTESIAN_POINT('Ctrl Pts',(15.6108257624088,3.30562953237115,-0.974596096350376));
#15565=CARTESIAN_POINT('Ctrl Pts',(15.3646843053979,3.33407731229027,-0.872325929581351));
#15566=CARTESIAN_POINT('Ctrl Pts',(15.2527291482116,3.3540348875684,-0.795495407366277));
#15567=CARTESIAN_POINT('Ctrl Pts',(15.0759748192914,3.39109395594973,-0.618741078446085));
#15568=CARTESIAN_POINT('Ctrl Pts',(14.9991265191444,3.41067812574963,-0.506776556958314));
#15569=CARTESIAN_POINT('Ctrl Pts',(14.8968432601511,3.43826042485992,-0.260601239755224));
#15570=CARTESIAN_POINT('Ctrl Pts',(14.8714473032184,3.44589712386029,-0.126333880758864));
#15571=CARTESIAN_POINT('Ctrl Pts',(14.8714473032184,3.44589712386029,-2.42861286636753E-16));
#15572=CARTESIAN_POINT('Ctrl Pts',(14.8714473032184,3.44589712386029,-1.38777878078145E-16));
#15573=CARTESIAN_POINT('Ctrl Pts',(14.8714473032184,3.44589712386029,0.126333880758864));
#15574=CARTESIAN_POINT('Ctrl Pts',(14.8968432601511,3.43826042485992,0.260601239755221));
#15575=CARTESIAN_POINT('Ctrl Pts',(14.9991265191444,3.41067812574963,0.506776556958312));
#15576=CARTESIAN_POINT('Ctrl Pts',(15.0759748192914,3.39109395594973,0.618741078446085));
#15577=CARTESIAN_POINT('Ctrl Pts',(15.2527291482116,3.3540348875684,0.795495407366277));
#15578=CARTESIAN_POINT('Ctrl Pts',(15.3646843053979,3.33407731229027,0.872325929581349));
#15579=CARTESIAN_POINT('Ctrl Pts',(15.6108257624088,3.30562953237115,0.974596096350375));
#15580=CARTESIAN_POINT('Ctrl Pts',(15.7450806494837,3.29760625124174,0.999999999999999));
#15581=CARTESIAN_POINT('Ctrl Pts',(15.8714473032184,3.29760625124174,0.999999999999999));
#15582=CARTESIAN_POINT('',(14.8714473032184,7.52312685038423,1.22464679914735E-16));
#15583=CARTESIAN_POINT('',(14.8714473032184,0.,1.22464679914735E-16));
#15584=CARTESIAN_POINT('',(15.8714473032184,7.45636892910833,0.999999999999999));
#15585=CARTESIAN_POINT('Ctrl Pts',(15.8714473032184,7.45636892910833,0.999999999999999));
#15586=CARTESIAN_POINT('Ctrl Pts',(15.7457245010652,7.45636892910833,0.999999999999999));
#15587=CARTESIAN_POINT('Ctrl Pts',(15.6117245964979,7.45987689127736,0.974843764196788));
#15588=CARTESIAN_POINT('Ctrl Pts',(15.3653900481838,7.47250970222183,0.872744136330349));
#15589=CARTESIAN_POINT('Ctrl Pts',(15.2530425360435,7.48144799782428,0.795808795198177));
#15590=CARTESIAN_POINT('Ctrl Pts',(15.0756394573932,7.49819644864561,0.618405716547907));
#15591=CARTESIAN_POINT('Ctrl Pts',(14.9987033720303,7.50710016352641,0.506057792670463));
#15592=CARTESIAN_POINT('Ctrl Pts',(14.8966032000273,7.51965370990447,0.259721846141313));
#15593=CARTESIAN_POINT('Ctrl Pts',(14.8714473032184,7.52312685038423,0.125721456548635));
#15594=CARTESIAN_POINT('Ctrl Pts',(14.8714473032184,7.52312685038423,-1.04083408558608E-16));
#15595=CARTESIAN_POINT('Ctrl Pts',(14.8714473032184,7.52312685038423,-2.08166817117217E-16));
#15596=CARTESIAN_POINT('Ctrl Pts',(14.8714473032184,7.52312685038423,-0.125721456548636));
#15597=CARTESIAN_POINT('Ctrl Pts',(14.8966032000273,7.51965370990447,-0.259721846141313));
#15598=CARTESIAN_POINT('Ctrl Pts',(14.9987033720303,7.50710016352641,-0.506057792670463));
#15599=CARTESIAN_POINT('Ctrl Pts',(15.0756394573932,7.49819644864561,-0.618405716547907));
#15600=CARTESIAN_POINT('Ctrl Pts',(15.2530425360435,7.48144799782428,-0.795808795198177));
#15601=CARTESIAN_POINT('Ctrl Pts',(15.3653900481838,7.47250970222183,-0.872744136330348));
#15602=CARTESIAN_POINT('Ctrl Pts',(15.6117245964979,7.45987689127736,-0.974843764196788));
#15603=CARTESIAN_POINT('Ctrl Pts',(15.7457245010652,7.45636892910833,-0.999999999999999));
#15604=CARTESIAN_POINT('Ctrl Pts',(15.9971701053716,7.45636892910833,-0.999999999999999));
#15605=CARTESIAN_POINT('Ctrl Pts',(16.1311700099389,7.45987689127736,-0.974843764196788));
#15606=CARTESIAN_POINT('Ctrl Pts',(16.377504558253,7.47250970222183,-0.872744136330349));
#15607=CARTESIAN_POINT('Ctrl Pts',(16.4898520703933,7.48144799782428,-0.795808795198177));
#15608=CARTESIAN_POINT('Ctrl Pts',(16.6672551490436,7.49819644864561,-0.618405716547907));
#15609=CARTESIAN_POINT('Ctrl Pts',(16.7441912344065,7.50710016352641,-0.506057792670463));
#15610=CARTESIAN_POINT('Ctrl Pts',(16.8462914064095,7.51965370990447,-0.259721846141313));
#15611=CARTESIAN_POINT('Ctrl Pts',(16.8714473032184,7.52312685038423,-0.125721456548635));
#15612=CARTESIAN_POINT('Ctrl Pts',(16.8714473032184,7.52312685038423,0.125721456548635));
#15613=CARTESIAN_POINT('Ctrl Pts',(16.8462914064095,7.51965370990447,0.259721846141313));
#15614=CARTESIAN_POINT('Ctrl Pts',(16.7441912344065,7.50710016352641,0.506057792670463));
#15615=CARTESIAN_POINT('Ctrl Pts',(16.6672551490436,7.49819644864561,0.618405716547907));
#15616=CARTESIAN_POINT('Ctrl Pts',(16.4898520703933,7.48144799782428,0.795808795198176));
#15617=CARTESIAN_POINT('Ctrl Pts',(16.377504558253,7.47250970222183,0.872744136330349));
#15618=CARTESIAN_POINT('Ctrl Pts',(16.1311700099389,7.45987689127736,0.974843764196788));
#15619=CARTESIAN_POINT('Ctrl Pts',(15.9971701053716,7.45636892910833,0.999999999999999));
#15620=CARTESIAN_POINT('Ctrl Pts',(15.8714473032184,7.45636892910833,0.999999999999999));
#15621=CARTESIAN_POINT('Origin',(11.0238490761438,0.,0.));
#15622=CARTESIAN_POINT('',(11.0238490761438,5.,-6.12323399573677E-16));
#15623=CARTESIAN_POINT('Origin',(11.0238490761438,0.,0.));
#15624=CARTESIAN_POINT('',(12.0767011645438,5.,-6.12323399573677E-16));
#15625=CARTESIAN_POINT('',(11.0238490761438,5.,6.12323399573677E-16));
#15626=CARTESIAN_POINT('Origin',(12.0767011645438,0.,0.));
#15627=CARTESIAN_POINT('Origin',(12.0767011645438,0.,0.));
#15628=CARTESIAN_POINT('',(12.076701164516,-4.22000688292658E-16,3.44589712386029));
#15629=CARTESIAN_POINT('Origin',(12.076701164516,0.,0.));
#15630=CARTESIAN_POINT('Origin',(11.474739121518,0.,0.));
#15631=CARTESIAN_POINT('',(11.9256291668923,-9.21317321690256E-16,7.52312685038423));
#15632=CARTESIAN_POINT('Origin',(11.9256291668923,0.,0.));
#15633=CARTESIAN_POINT('',(11.0238490761438,-8.44001376585316E-16,6.89179424772059));
#15634=CARTESIAN_POINT('',(11.474739121518,-8.82659349137786E-16,7.20746054905241));
#15635=CARTESIAN_POINT('Origin',(11.0238490761438,0.,0.));
#15636=CARTESIAN_POINT('Origin',(16.3019119808107,0.,0.));
#15637=CARTESIAN_POINT('',(20.6781947947292,-9.21317321690256E-16,7.52312685038423));
#15638=CARTESIAN_POINT('Origin',(20.6781947947292,0.,0.));
#15639=CARTESIAN_POINT('',(16.3019119808107,-9.21317321690256E-16,7.52312685038423));
#15640=CARTESIAN_POINT('Origin',(20.9315098273138,0.,0.));
#15641=CARTESIAN_POINT('',(21.1848248598985,-8.82659349137786E-16,7.20746054905241));
#15642=CARTESIAN_POINT('',(20.9315098273138,9.01988335414021E-16,7.36529369971832));
#15643=CARTESIAN_POINT('Origin',(21.1848248598985,0.,0.));
#15644=CARTESIAN_POINT('Origin',(21.4140009475395,0.,0.));
#15645=CARTESIAN_POINT('',(21.4140009475395,-9.02308225835327E-16,7.36790580323689));
#15646=CARTESIAN_POINT('Origin',(53.9616500647475,0.,0.));
#15647=CARTESIAN_POINT('',(31.6525499953511,-7.84960767273423E-16,6.40969108660508));
#15648=CARTESIAN_POINT('Origin',(31.6525499953511,0.,0.));
#15649=CARTESIAN_POINT('',(53.9616500647475,-7.85768394580416E-16,6.41628586403442));
#15650=CARTESIAN_POINT('Origin',(31.0318089645314,0.,0.));
#15651=CARTESIAN_POINT('',(30.4110679337117,-7.84960767273423E-16,6.40969108660508));
#15652=CARTESIAN_POINT('Origin',(30.4110679337117,0.,0.));
#15653=CARTESIAN_POINT('',(31.0318089645314,-7.84960767273423E-16,6.40969108660508));
#15654=CARTESIAN_POINT('Origin',(29.5420239984498,0.,0.));
#15655=CARTESIAN_POINT('',(28.6729800631879,-7.84852901782084E-16,6.40881029802658));
#15656=CARTESIAN_POINT('Origin',(28.6729800631879,0.,0.));
#15657=CARTESIAN_POINT('',(29.5420239984498,-7.84884362648318E-16,6.40906719549494));
#15658=CARTESIAN_POINT('Origin',(28.6729800631879,0.,-6.41550316824698));
#15659=CARTESIAN_POINT('',(28.6729800631879,-7.85672541991337E-16,6.41550316824698));
#15660=CARTESIAN_POINT('Origin',(28.6729800631879,0.,0.));
#15661=CARTESIAN_POINT('Origin',(28.2136282688352,0.,0.));
#15662=CARTESIAN_POINT('',(27.7542764744824,-7.85672541991337E-16,6.41550316824698));
#15663=CARTESIAN_POINT('Origin',(27.7542764744824,0.,0.));
#15664=CARTESIAN_POINT('',(28.2136282688352,-7.85672541991337E-16,6.41550316824698));
#15665=CARTESIAN_POINT('Origin',(27.7542764744824,0.,-6.40853872070288));
#15666=CARTESIAN_POINT('',(27.7542764744824,-7.84819643152065E-16,6.40853872070288));
#15667=CARTESIAN_POINT('Origin',(27.7542764744824,0.,0.));
#15668=CARTESIAN_POINT('Origin',(26.6245076505395,0.,0.));
#15669=CARTESIAN_POINT('',(25.4947388265965,-7.84737844052149E-16,6.40787078036307));
#15670=CARTESIAN_POINT('Origin',(25.4947388265965,0.,0.));
#15671=CARTESIAN_POINT('',(26.6245076505395,-7.84778743602106E-16,6.40820475053297));
#15672=CARTESIAN_POINT('Origin',(25.0105689136245,0.,0.));
#15673=CARTESIAN_POINT('',(24.5263990006525,-7.84737844052149E-16,6.40787078036307));
#15674=CARTESIAN_POINT('Origin',(24.5263990006525,0.,0.));
#15675=CARTESIAN_POINT('',(25.0105689136245,-7.84737844052149E-16,6.40787078036307));
#15676=CARTESIAN_POINT('Origin',(23.6497386319918,0.,0.));
#15677=CARTESIAN_POINT('',(22.7730782633312,-7.84639315317936E-16,6.40706623219228));
#15678=CARTESIAN_POINT('Origin',(22.7730782633312,0.,0.));
#15679=CARTESIAN_POINT('',(23.6497386319918,-7.84671051911994E-16,6.40732538114918));
#15680=CARTESIAN_POINT('Origin',(22.2310089528171,0.,0.));
#15681=CARTESIAN_POINT('',(21.688939642303,-7.84639315317937E-16,6.40706623219228));
#15682=CARTESIAN_POINT('Origin',(21.688939642303,0.,0.));
#15683=CARTESIAN_POINT('',(22.2310089528171,-7.84639315317937E-16,6.40706623219228));
#15684=CARTESIAN_POINT('Origin',(21.4368822511007,0.,0.));
#15685=CARTESIAN_POINT('',(21.1848248598985,-7.8458181784762E-16,6.4065967297173));
#15686=CARTESIAN_POINT('Origin',(21.1848248598985,0.,0.));
#15687=CARTESIAN_POINT('',(21.4368822511007,-7.84590942753216E-16,6.40667124022599));
#15688=CARTESIAN_POINT('Origin',(21.1848248598985,0.,-4.66385643997278));
#15689=CARTESIAN_POINT('',(21.1848248598985,-5.71157686089543E-16,4.66385643997278));
#15690=CARTESIAN_POINT('Origin',(21.1848248598985,0.,0.));
#15691=CARTESIAN_POINT('Origin',(20.4983944566926,0.,0.));
#15692=CARTESIAN_POINT('',(19.8119640534868,-5.71157686089543E-16,4.66385643997278));
#15693=CARTESIAN_POINT('Origin',(19.8119640534868,0.,0.));
#15694=CARTESIAN_POINT('',(20.4983944566926,-5.71157686089543E-16,4.66385643997278));
#15695=CARTESIAN_POINT('Origin',(19.8119640534868,0.,-3.44589712386029));
#15696=CARTESIAN_POINT('',(19.8119640534868,-4.22000688292658E-16,3.44589712386029));
#15697=CARTESIAN_POINT('Origin',(19.8119640534868,0.,0.));
#15698=CARTESIAN_POINT('Origin',(15.9443326090014,0.,0.));
#15699=CARTESIAN_POINT('',(15.9443326090014,-4.22000688292657E-16,3.44589712386029));
#15700=CARTESIAN_POINT('Origin',(11.0238490761438,0.,-6.89179424772059));
#27691=UNCERTAINTY_MEASURE_WITH_UNIT(LENGTH_MEASURE(0.01),#27708,
'DISTANCE_ACCURACY_VALUE',
'Maximum model space distance between geometric entities at asserted c
onnectivities');
#27695=UNCERTAINTY_MEASURE_WITH_UNIT(LENGTH_MEASURE(0.01),#27708,
'DISTANCE_ACCURACY_VALUE',
'Maximum model space distance between geometric entities at asserted c
onnectivities');
#27703=(
GEOMETRIC_REPRESENTATION_CONTEXT(3)
GLOBAL_UNCERTAINTY_ASSIGNED_CONTEXT((#27691))
GLOBAL_UNIT_ASSIGNED_CONTEXT((#27708,#27710,#27711))
REPRESENTATION_CONTEXT('','3D')
);
#27707=(
GEOMETRIC_REPRESENTATION_CONTEXT(3)
GLOBAL_UNCERTAINTY_ASSIGNED_CONTEXT((#27695))
GLOBAL_UNIT_ASSIGNED_CONTEXT((#27708,#27710,#27711))
REPRESENTATION_CONTEXT('','3D')
);
#27708=(
LENGTH_UNIT()
NAMED_UNIT(*)
SI_UNIT(.MILLI.,.METRE.)
);
#27710=(
NAMED_UNIT(*)
PLANE_ANGLE_UNIT()
SI_UNIT($,.RADIAN.)
);
#27711=(
NAMED_UNIT(*)
SI_UNIT($,.STERADIAN.)
SOLID_ANGLE_UNIT()
);
#27719=SHAPE_DEFINITION_REPRESENTATION(#27730,#27751);
#27730=PRODUCT_DEFINITION_SHAPE('',$,#27763);
#27751=SHAPE_REPRESENTATION('',(#4092),#27703);
#27755=PRODUCT_DEFINITION_CONTEXT('part definition',#27790,'design');
#27763=PRODUCT_DEFINITION('Cylinder','Cylinder',#27774,#27755);
#27774=PRODUCT_DEFINITION_FORMATION('',$,#27799);
#27790=APPLICATION_CONTEXT(
'Core Data for Automotive Mechanical Design Process');
#27791=PRODUCT_CONTEXT('part definition',#27790,'mechanical');
#27799=PRODUCT('Cylinder','Cylinder',$,(#27791));
#27804=PRESENTATION_STYLE_ASSIGNMENT((#27806));
#27806=SURFACE_STYLE_USAGE(.BOTH.,#27808);
#27808=SURFACE_SIDE_STYLE('',(#27810));
#27810=SURFACE_STYLE_FILL_AREA(#27812);
#27812=FILL_AREA_STYLE('Opaque(160,160,160)',(#27814));
#27814=FILL_AREA_STYLE_COLOUR('Opaque(160,160,160)',#27816);
#27816=COLOUR_RGB('Opaque(160,160,160)', 0.09019608, 0.27058824, 0.51372549);
ENDSEC;
END-ISO-10303-21;
